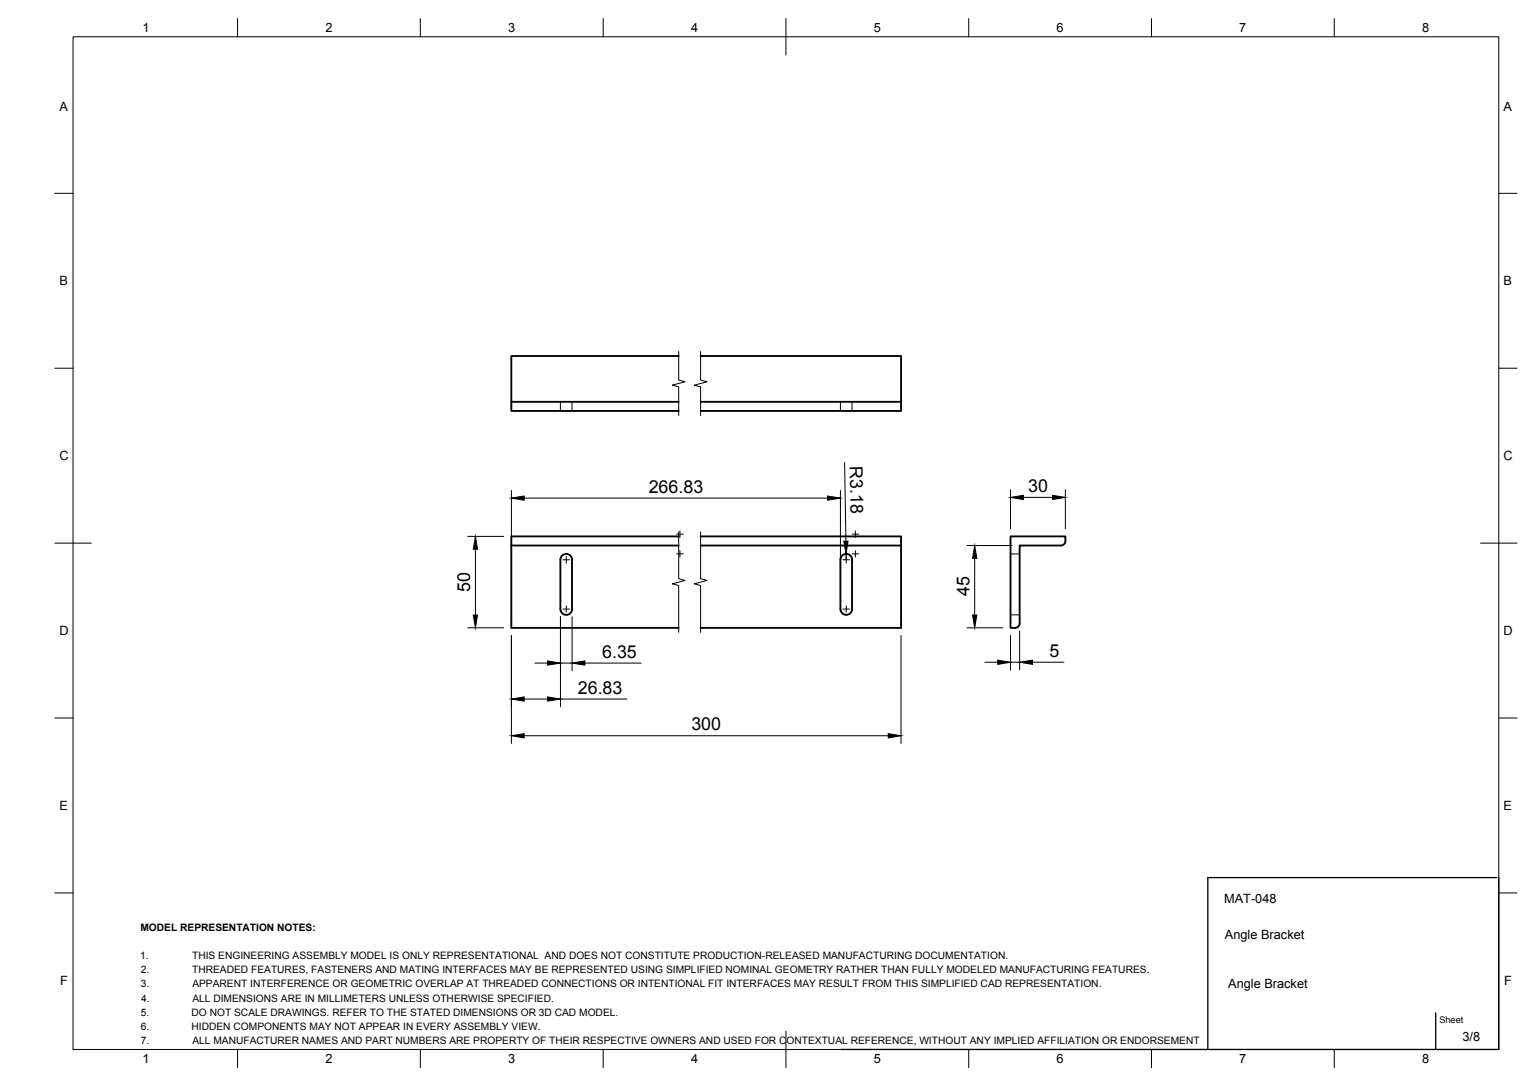
ISO-10303-21;
HEADER;
/* Generated by software containing ST-Developer
 * from STEP Tools, Inc. (www.steptools.com) 
 */

FILE_DESCRIPTION(
/* description */ ('STEP AP214'),
/* implementation_level */ '2;1');

FILE_NAME(
/* name */ 'Angle Bracket.step',
/* time_stamp */ '2026-11-14T22:24:45-08:00',
/* author */ (''),
/* organization */ (''),
/* preprocessor_version */ 'ST-DEVELOPER v20.2',
/* originating_system */ 'Autodesk Translation Framework v15.17.0.0',
/* authorisation */ '');

FILE_SCHEMA (('AUTOMOTIVE_DESIGN { 1 0 10303 214 3 1 1 }'));
ENDSEC;

DATA;
#10=MECHANICAL_DESIGN_GEOMETRIC_PRESENTATION_REPRESENTATION('',(#127),#5599);
#99=FACE_BOUND('',#563,.T.);
#100=FACE_BOUND('',#564,.T.);
#101=FACE_BOUND('',#570,.T.);
#102=FACE_BOUND('',#571,.T.);
#115=SHAPE_REPRESENTATION_RELATIONSHIP('SRR','None',#5643,#121);
#121=ADVANCED_BREP_SHAPE_REPRESENTATION('',(#133),#5595);
#127=STYLED_ITEM('',(#5681),#133);
#133=MANIFOLD_SOLID_BREP('Body1',#3309);
#165=CYLINDRICAL_SURFACE('',#3536,2.5);
#166=CYLINDRICAL_SURFACE('',#3545,2.5);
#167=CYLINDRICAL_SURFACE('',#3550,3.17499999999993);
#168=CYLINDRICAL_SURFACE('',#3552,3.17499999999993);
#169=CYLINDRICAL_SURFACE('',#3554,3.17499999999993);
#170=CYLINDRICAL_SURFACE('',#3556,3.17499999999993);
#225=CIRCLE('',#3530,3.17499999999993);
#226=CIRCLE('',#3531,3.17499999999993);
#227=CIRCLE('',#3532,3.17499999999993);
#228=CIRCLE('',#3533,3.17499999999993);
#229=CIRCLE('',#3537,2.5);
#230=CIRCLE('',#3538,2.5);
#231=CIRCLE('',#3541,3.17499999999993);
#232=CIRCLE('',#3542,3.17499999999993);
#233=CIRCLE('',#3543,3.17499999999993);
#234=CIRCLE('',#3544,3.17499999999993);
#235=CIRCLE('',#3546,2.5);
#236=CIRCLE('',#3547,2.5);
#385=FACE_OUTER_BOUND('',#561,.T.);
#386=FACE_OUTER_BOUND('',#562,.T.);
#387=FACE_OUTER_BOUND('',#565,.T.);
#388=FACE_OUTER_BOUND('',#566,.T.);
#389=FACE_OUTER_BOUND('',#567,.T.);
#390=FACE_OUTER_BOUND('',#568,.T.);
#391=FACE_OUTER_BOUND('',#569,.T.);
#392=FACE_OUTER_BOUND('',#572,.T.);
#393=FACE_OUTER_BOUND('',#573,.T.);
#394=FACE_OUTER_BOUND('',#574,.T.);
#395=FACE_OUTER_BOUND('',#575,.T.);
#396=FACE_OUTER_BOUND('',#576,.T.);
#397=FACE_OUTER_BOUND('',#577,.T.);
#398=FACE_OUTER_BOUND('',#578,.T.);
#399=FACE_OUTER_BOUND('',#579,.T.);
#400=FACE_OUTER_BOUND('',#580,.T.);
#401=FACE_OUTER_BOUND('',#581,.T.);
#402=FACE_OUTER_BOUND('',#582,.T.);
#561=EDGE_LOOP('',(#2635,#2636,#2637,#2638));
#562=EDGE_LOOP('',(#2639,#2640,#2641,#2642));
#563=EDGE_LOOP('',(#2643,#2644,#2645,#2646));
#564=EDGE_LOOP('',(#2647,#2648,#2649,#2650));
#565=EDGE_LOOP('',(#2651,#2652,#2653,#2654));
#566=EDGE_LOOP('',(#2655,#2656,#2657,#2658));
#567=EDGE_LOOP('',(#2659,#2660,#2661,#2662));
#568=EDGE_LOOP('',(#2663,#2664,#2665,#2666));
#569=EDGE_LOOP('',(#2667,#2668,#2669,#2670));
#570=EDGE_LOOP('',(#2671,#2672,#2673,#2674));
#571=EDGE_LOOP('',(#2675,#2676,#2677,#2678));
#572=EDGE_LOOP('',(#2679,#2680,#2681,#2682));
#573=EDGE_LOOP('',(#2683,#2684,#2685,#2686,#2687,#2688,#2689,#2690));
#574=EDGE_LOOP('',(#2691,#2692,#2693,#2694,#2695,#2696,#2697,#2698));
#575=EDGE_LOOP('',(#2699,#2700,#2701,#2702));
#576=EDGE_LOOP('',(#2703,#2704,#2705,#2706));
#577=EDGE_LOOP('',(#2707,#2708,#2709,#2710));
#578=EDGE_LOOP('',(#2711,#2712,#2713,#2714));
#579=EDGE_LOOP('',(#2715,#2716,#2717,#2718));
#580=EDGE_LOOP('',(#2719,#2720,#2721,#2722));
#581=EDGE_LOOP('',(#2723,#2724,#2725,#2726));
#582=EDGE_LOOP('',(#2727,#2728,#2729,#2730));
#875=LINE('',#5186,#1231);
#876=LINE('',#5188,#1232);
#877=LINE('',#5190,#1233);
#878=LINE('',#5191,#1234);
#879=LINE('',#5194,#1235);
#880=LINE('',#5196,#1236);
#881=LINE('',#5197,#1237);
#882=LINE('',#5200,#1238);
#883=LINE('',#5204,#1239);
#884=LINE('',#5208,#1240);
#885=LINE('',#5212,#1241);
#886=LINE('',#5216,#1242);
#887=LINE('',#5218,#1243);
#888=LINE('',#5219,#1244);
#889=LINE('',#5222,#1245);
#890=LINE('',#5224,#1246);
#891=LINE('',#5225,#1247);
#892=LINE('',#5230,#1248);
#893=LINE('',#5234,#1249);
#894=LINE('',#5236,#1250);
#895=LINE('',#5237,#1251);
#896=LINE('',#5240,#1252);
#897=LINE('',#5242,#1253);
#898=LINE('',#5243,#1254);
#899=LINE('',#5246,#1255);
#900=LINE('',#5250,#1256);
#901=LINE('',#5254,#1257);
#902=LINE('',#5258,#1258);
#903=LINE('',#5266,#1259);
#904=LINE('',#5267,#1260);
#905=LINE('',#5269,#1261);
#906=LINE('',#5271,#1262);
#907=LINE('',#5274,#1263);
#908=LINE('',#5275,#1264);
#909=LINE('',#5277,#1265);
#910=LINE('',#5279,#1266);
#1231=VECTOR('',#4207,1000.);
#1232=VECTOR('',#4208,1000.);
#1233=VECTOR('',#4209,1000.);
#1234=VECTOR('',#4210,1000.);
#1235=VECTOR('',#4213,1000.);
#1236=VECTOR('',#4214,1000.);
#1237=VECTOR('',#4215,1000.);
#1238=VECTOR('',#4216,1000.);
#1239=VECTOR('',#4219,1000.);
#1240=VECTOR('',#4222,1000.);
#1241=VECTOR('',#4225,1000.);
#1242=VECTOR('',#4230,1000.);
#1243=VECTOR('',#4231,1000.);
#1244=VECTOR('',#4232,1000.);
#1245=VECTOR('',#4235,1000.);
#1246=VECTOR('',#4236,1000.);
#1247=VECTOR('',#4237,1000.);
#1248=VECTOR('',#4242,1000.);
#1249=VECTOR('',#4247,1000.);
#1250=VECTOR('',#4248,1000.);
#1251=VECTOR('',#4249,1000.);
#1252=VECTOR('',#4252,1000.);
#1253=VECTOR('',#4253,1000.);
#1254=VECTOR('',#4254,1000.);
#1255=VECTOR('',#4255,1000.);
#1256=VECTOR('',#4258,1000.);
#1257=VECTOR('',#4261,1000.);
#1258=VECTOR('',#4264,1000.);
#1259=VECTOR('',#4279,1000.);
#1260=VECTOR('',#4280,1000.);
#1261=VECTOR('',#4283,1000.);
#1262=VECTOR('',#4286,1000.);
#1263=VECTOR('',#4291,1000.);
#1264=VECTOR('',#4292,1000.);
#1265=VECTOR('',#4295,1000.);
#1266=VECTOR('',#4298,1000.);
#1527=VERTEX_POINT('',#5184);
#1528=VERTEX_POINT('',#5185);
#1529=VERTEX_POINT('',#5187);
#1530=VERTEX_POINT('',#5189);
#1531=VERTEX_POINT('',#5193);
#1532=VERTEX_POINT('',#5195);
#1533=VERTEX_POINT('',#5198);
#1534=VERTEX_POINT('',#5199);
#1535=VERTEX_POINT('',#5201);
#1536=VERTEX_POINT('',#5203);
#1537=VERTEX_POINT('',#5206);
#1538=VERTEX_POINT('',#5207);
#1539=VERTEX_POINT('',#5209);
#1540=VERTEX_POINT('',#5211);
#1541=VERTEX_POINT('',#5215);
#1542=VERTEX_POINT('',#5217);
#1543=VERTEX_POINT('',#5221);
#1544=VERTEX_POINT('',#5223);
#1545=VERTEX_POINT('',#5227);
#1546=VERTEX_POINT('',#5229);
#1547=VERTEX_POINT('',#5233);
#1548=VERTEX_POINT('',#5235);
#1549=VERTEX_POINT('',#5239);
#1550=VERTEX_POINT('',#5241);
#1551=VERTEX_POINT('',#5244);
#1552=VERTEX_POINT('',#5245);
#1553=VERTEX_POINT('',#5247);
#1554=VERTEX_POINT('',#5249);
#1555=VERTEX_POINT('',#5252);
#1556=VERTEX_POINT('',#5253);
#1557=VERTEX_POINT('',#5255);
#1558=VERTEX_POINT('',#5257);
#1915=EDGE_CURVE('',#1527,#1528,#875,.T.);
#1916=EDGE_CURVE('',#1529,#1528,#876,.T.);
#1917=EDGE_CURVE('',#1530,#1529,#877,.T.);
#1918=EDGE_CURVE('',#1530,#1527,#878,.T.);
#1919=EDGE_CURVE('',#1528,#1531,#879,.T.);
#1920=EDGE_CURVE('',#1532,#1531,#880,.T.);
#1921=EDGE_CURVE('',#1529,#1532,#881,.T.);
#1922=EDGE_CURVE('',#1533,#1534,#882,.T.);
#1923=EDGE_CURVE('',#1534,#1535,#225,.T.);
#1924=EDGE_CURVE('',#1535,#1536,#883,.T.);
#1925=EDGE_CURVE('',#1536,#1533,#226,.T.);
#1926=EDGE_CURVE('',#1537,#1538,#884,.T.);
#1927=EDGE_CURVE('',#1538,#1539,#227,.T.);
#1928=EDGE_CURVE('',#1539,#1540,#885,.T.);
#1929=EDGE_CURVE('',#1540,#1537,#228,.T.);
#1930=EDGE_CURVE('',#1531,#1541,#886,.T.);
#1931=EDGE_CURVE('',#1542,#1541,#887,.T.);
#1932=EDGE_CURVE('',#1532,#1542,#888,.T.);
#1933=EDGE_CURVE('',#1541,#1543,#889,.T.);
#1934=EDGE_CURVE('',#1544,#1543,#890,.T.);
#1935=EDGE_CURVE('',#1542,#1544,#891,.T.);
#1936=EDGE_CURVE('',#1543,#1545,#229,.T.);
#1937=EDGE_CURVE('',#1546,#1545,#892,.T.);
#1938=EDGE_CURVE('',#1544,#1546,#230,.T.);
#1939=EDGE_CURVE('',#1545,#1547,#893,.T.);
#1940=EDGE_CURVE('',#1548,#1547,#894,.T.);
#1941=EDGE_CURVE('',#1546,#1548,#895,.T.);
#1942=EDGE_CURVE('',#1547,#1549,#896,.T.);
#1943=EDGE_CURVE('',#1550,#1549,#897,.T.);
#1944=EDGE_CURVE('',#1548,#1550,#898,.T.);
#1945=EDGE_CURVE('',#1551,#1552,#899,.T.);
#1946=EDGE_CURVE('',#1553,#1551,#231,.T.);
#1947=EDGE_CURVE('',#1554,#1553,#900,.T.);
#1948=EDGE_CURVE('',#1552,#1554,#232,.T.);
#1949=EDGE_CURVE('',#1555,#1556,#901,.T.);
#1950=EDGE_CURVE('',#1557,#1555,#233,.T.);
#1951=EDGE_CURVE('',#1558,#1557,#902,.T.);
#1952=EDGE_CURVE('',#1556,#1558,#234,.T.);
#1953=EDGE_CURVE('',#1549,#1527,#235,.T.);
#1954=EDGE_CURVE('',#1550,#1530,#236,.T.);
#1955=EDGE_CURVE('',#1538,#1557,#903,.T.);
#1956=EDGE_CURVE('',#1539,#1555,#904,.T.);
#1957=EDGE_CURVE('',#1537,#1558,#905,.T.);
#1958=EDGE_CURVE('',#1540,#1556,#906,.T.);
#1959=EDGE_CURVE('',#1534,#1553,#907,.T.);
#1960=EDGE_CURVE('',#1535,#1551,#908,.T.);
#1961=EDGE_CURVE('',#1533,#1554,#909,.T.);
#1962=EDGE_CURVE('',#1536,#1552,#910,.T.);
#2635=ORIENTED_EDGE('',*,*,#1915,.T.);
#2636=ORIENTED_EDGE('',*,*,#1916,.F.);
#2637=ORIENTED_EDGE('',*,*,#1917,.F.);
#2638=ORIENTED_EDGE('',*,*,#1918,.T.);
#2639=ORIENTED_EDGE('',*,*,#1919,.T.);
#2640=ORIENTED_EDGE('',*,*,#1920,.F.);
#2641=ORIENTED_EDGE('',*,*,#1921,.F.);
#2642=ORIENTED_EDGE('',*,*,#1916,.T.);
#2643=ORIENTED_EDGE('',*,*,#1922,.T.);
#2644=ORIENTED_EDGE('',*,*,#1923,.T.);
#2645=ORIENTED_EDGE('',*,*,#1924,.T.);
#2646=ORIENTED_EDGE('',*,*,#1925,.T.);
#2647=ORIENTED_EDGE('',*,*,#1926,.T.);
#2648=ORIENTED_EDGE('',*,*,#1927,.T.);
#2649=ORIENTED_EDGE('',*,*,#1928,.T.);
#2650=ORIENTED_EDGE('',*,*,#1929,.T.);
#2651=ORIENTED_EDGE('',*,*,#1930,.T.);
#2652=ORIENTED_EDGE('',*,*,#1931,.F.);
#2653=ORIENTED_EDGE('',*,*,#1932,.F.);
#2654=ORIENTED_EDGE('',*,*,#1920,.T.);
#2655=ORIENTED_EDGE('',*,*,#1933,.T.);
#2656=ORIENTED_EDGE('',*,*,#1934,.F.);
#2657=ORIENTED_EDGE('',*,*,#1935,.F.);
#2658=ORIENTED_EDGE('',*,*,#1931,.T.);
#2659=ORIENTED_EDGE('',*,*,#1936,.T.);
#2660=ORIENTED_EDGE('',*,*,#1937,.F.);
#2661=ORIENTED_EDGE('',*,*,#1938,.F.);
#2662=ORIENTED_EDGE('',*,*,#1934,.T.);
#2663=ORIENTED_EDGE('',*,*,#1939,.T.);
#2664=ORIENTED_EDGE('',*,*,#1940,.F.);
#2665=ORIENTED_EDGE('',*,*,#1941,.F.);
#2666=ORIENTED_EDGE('',*,*,#1937,.T.);
#2667=ORIENTED_EDGE('',*,*,#1942,.T.);
#2668=ORIENTED_EDGE('',*,*,#1943,.F.);
#2669=ORIENTED_EDGE('',*,*,#1944,.F.);
#2670=ORIENTED_EDGE('',*,*,#1940,.T.);
#2671=ORIENTED_EDGE('',*,*,#1945,.F.);
#2672=ORIENTED_EDGE('',*,*,#1946,.F.);
#2673=ORIENTED_EDGE('',*,*,#1947,.F.);
#2674=ORIENTED_EDGE('',*,*,#1948,.F.);
#2675=ORIENTED_EDGE('',*,*,#1949,.F.);
#2676=ORIENTED_EDGE('',*,*,#1950,.F.);
#2677=ORIENTED_EDGE('',*,*,#1951,.F.);
#2678=ORIENTED_EDGE('',*,*,#1952,.F.);
#2679=ORIENTED_EDGE('',*,*,#1953,.T.);
#2680=ORIENTED_EDGE('',*,*,#1918,.F.);
#2681=ORIENTED_EDGE('',*,*,#1954,.F.);
#2682=ORIENTED_EDGE('',*,*,#1943,.T.);
#2683=ORIENTED_EDGE('',*,*,#1917,.T.);
#2684=ORIENTED_EDGE('',*,*,#1921,.T.);
#2685=ORIENTED_EDGE('',*,*,#1932,.T.);
#2686=ORIENTED_EDGE('',*,*,#1935,.T.);
#2687=ORIENTED_EDGE('',*,*,#1938,.T.);
#2688=ORIENTED_EDGE('',*,*,#1941,.T.);
#2689=ORIENTED_EDGE('',*,*,#1944,.T.);
#2690=ORIENTED_EDGE('',*,*,#1954,.T.);
#2691=ORIENTED_EDGE('',*,*,#1915,.F.);
#2692=ORIENTED_EDGE('',*,*,#1953,.F.);
#2693=ORIENTED_EDGE('',*,*,#1942,.F.);
#2694=ORIENTED_EDGE('',*,*,#1939,.F.);
#2695=ORIENTED_EDGE('',*,*,#1936,.F.);
#2696=ORIENTED_EDGE('',*,*,#1933,.F.);
#2697=ORIENTED_EDGE('',*,*,#1930,.F.);
#2698=ORIENTED_EDGE('',*,*,#1919,.F.);
#2699=ORIENTED_EDGE('',*,*,#1955,.T.);
#2700=ORIENTED_EDGE('',*,*,#1950,.T.);
#2701=ORIENTED_EDGE('',*,*,#1956,.F.);
#2702=ORIENTED_EDGE('',*,*,#1927,.F.);
#2703=ORIENTED_EDGE('',*,*,#1957,.T.);
#2704=ORIENTED_EDGE('',*,*,#1951,.T.);
#2705=ORIENTED_EDGE('',*,*,#1955,.F.);
#2706=ORIENTED_EDGE('',*,*,#1926,.F.);
#2707=ORIENTED_EDGE('',*,*,#1958,.T.);
#2708=ORIENTED_EDGE('',*,*,#1952,.T.);
#2709=ORIENTED_EDGE('',*,*,#1957,.F.);
#2710=ORIENTED_EDGE('',*,*,#1929,.F.);
#2711=ORIENTED_EDGE('',*,*,#1956,.T.);
#2712=ORIENTED_EDGE('',*,*,#1949,.T.);
#2713=ORIENTED_EDGE('',*,*,#1958,.F.);
#2714=ORIENTED_EDGE('',*,*,#1928,.F.);
#2715=ORIENTED_EDGE('',*,*,#1959,.T.);
#2716=ORIENTED_EDGE('',*,*,#1946,.T.);
#2717=ORIENTED_EDGE('',*,*,#1960,.F.);
#2718=ORIENTED_EDGE('',*,*,#1923,.F.);
#2719=ORIENTED_EDGE('',*,*,#1961,.T.);
#2720=ORIENTED_EDGE('',*,*,#1947,.T.);
#2721=ORIENTED_EDGE('',*,*,#1959,.F.);
#2722=ORIENTED_EDGE('',*,*,#1922,.F.);
#2723=ORIENTED_EDGE('',*,*,#1962,.T.);
#2724=ORIENTED_EDGE('',*,*,#1948,.T.);
#2725=ORIENTED_EDGE('',*,*,#1961,.F.);
#2726=ORIENTED_EDGE('',*,*,#1925,.F.);
#2727=ORIENTED_EDGE('',*,*,#1960,.T.);
#2728=ORIENTED_EDGE('',*,*,#1945,.T.);
#2729=ORIENTED_EDGE('',*,*,#1962,.F.);
#2730=ORIENTED_EDGE('',*,*,#1924,.F.);
#3087=PLANE('',#3528);
#3088=PLANE('',#3529);
#3089=PLANE('',#3534);
#3090=PLANE('',#3535);
#3091=PLANE('',#3539);
#3092=PLANE('',#3540);
#3093=PLANE('',#3548);
#3094=PLANE('',#3549);
#3095=PLANE('',#3551);
#3096=PLANE('',#3553);
#3097=PLANE('',#3555);
#3098=PLANE('',#3557);
#3235=ADVANCED_FACE('',(#385),#3087,.F.);
#3236=ADVANCED_FACE('',(#386,#99,#100),#3088,.F.);
#3237=ADVANCED_FACE('',(#387),#3089,.F.);
#3238=ADVANCED_FACE('',(#388),#3090,.F.);
#3239=ADVANCED_FACE('',(#389),#165,.T.);
#3240=ADVANCED_FACE('',(#390),#3091,.F.);
#3241=ADVANCED_FACE('',(#391,#101,#102),#3092,.F.);
#3242=ADVANCED_FACE('',(#392),#166,.T.);
#3243=ADVANCED_FACE('',(#393),#3093,.T.);
#3244=ADVANCED_FACE('',(#394),#3094,.F.);
#3245=ADVANCED_FACE('',(#395),#167,.F.);
#3246=ADVANCED_FACE('',(#396),#3095,.F.);
#3247=ADVANCED_FACE('',(#397),#168,.F.);
#3248=ADVANCED_FACE('',(#398),#3096,.F.);
#3249=ADVANCED_FACE('',(#399),#169,.F.);
#3250=ADVANCED_FACE('',(#400),#3097,.F.);
#3251=ADVANCED_FACE('',(#401),#170,.F.);
#3252=ADVANCED_FACE('',(#402),#3098,.F.);
#3309=CLOSED_SHELL('',(#3235,#3236,#3237,#3238,#3239,#3240,#3241,#3242,
#3243,#3244,#3245,#3246,#3247,#3248,#3249,#3250,#3251,#3252));
#3527=AXIS2_PLACEMENT_3D('',#5182,#4203,#4204);
#3528=AXIS2_PLACEMENT_3D('',#5183,#4205,#4206);
#3529=AXIS2_PLACEMENT_3D('',#5192,#4211,#4212);
#3530=AXIS2_PLACEMENT_3D('',#5202,#4217,#4218);
#3531=AXIS2_PLACEMENT_3D('',#5205,#4220,#4221);
#3532=AXIS2_PLACEMENT_3D('',#5210,#4223,#4224);
#3533=AXIS2_PLACEMENT_3D('',#5213,#4226,#4227);
#3534=AXIS2_PLACEMENT_3D('',#5214,#4228,#4229);
#3535=AXIS2_PLACEMENT_3D('',#5220,#4233,#4234);
#3536=AXIS2_PLACEMENT_3D('',#5226,#4238,#4239);
#3537=AXIS2_PLACEMENT_3D('',#5228,#4240,#4241);
#3538=AXIS2_PLACEMENT_3D('',#5231,#4243,#4244);
#3539=AXIS2_PLACEMENT_3D('',#5232,#4245,#4246);
#3540=AXIS2_PLACEMENT_3D('',#5238,#4250,#4251);
#3541=AXIS2_PLACEMENT_3D('',#5248,#4256,#4257);
#3542=AXIS2_PLACEMENT_3D('',#5251,#4259,#4260);
#3543=AXIS2_PLACEMENT_3D('',#5256,#4262,#4263);
#3544=AXIS2_PLACEMENT_3D('',#5259,#4265,#4266);
#3545=AXIS2_PLACEMENT_3D('',#5260,#4267,#4268);
#3546=AXIS2_PLACEMENT_3D('',#5261,#4269,#4270);
#3547=AXIS2_PLACEMENT_3D('',#5262,#4271,#4272);
#3548=AXIS2_PLACEMENT_3D('',#5263,#4273,#4274);
#3549=AXIS2_PLACEMENT_3D('',#5264,#4275,#4276);
#3550=AXIS2_PLACEMENT_3D('',#5265,#4277,#4278);
#3551=AXIS2_PLACEMENT_3D('',#5268,#4281,#4282);
#3552=AXIS2_PLACEMENT_3D('',#5270,#4284,#4285);
#3553=AXIS2_PLACEMENT_3D('',#5272,#4287,#4288);
#3554=AXIS2_PLACEMENT_3D('',#5273,#4289,#4290);
#3555=AXIS2_PLACEMENT_3D('',#5276,#4293,#4294);
#3556=AXIS2_PLACEMENT_3D('',#5278,#4296,#4297);
#3557=AXIS2_PLACEMENT_3D('',#5280,#4299,#4300);
#4203=DIRECTION('axis',(0.,0.,1.));
#4204=DIRECTION('refdir',(1.,0.,0.));
#4205=DIRECTION('center_axis',(1.,0.,0.));
#4206=DIRECTION('ref_axis',(0.,0.,-1.));
#4207=DIRECTION('',(0.,-1.,0.));
#4208=DIRECTION('',(0.,0.,-1.));
#4209=DIRECTION('',(0.,-1.,0.));
#4210=DIRECTION('',(0.,0.,-1.));
#4211=DIRECTION('center_axis',(0.,1.,0.));
#4212=DIRECTION('ref_axis',(0.,0.,1.));
#4213=DIRECTION('',(1.,0.,0.));
#4214=DIRECTION('',(0.,0.,-1.));
#4215=DIRECTION('',(1.,0.,0.));
#4216=DIRECTION('',(-1.,0.,1.28577838368676E-16));
#4217=DIRECTION('center_axis',(0.,1.,0.));
#4218=DIRECTION('ref_axis',(0.,0.,1.));
#4219=DIRECTION('',(1.,0.,0.));
#4220=DIRECTION('center_axis',(0.,1.,0.));
#4221=DIRECTION('ref_axis',(0.,0.,1.));
#4222=DIRECTION('',(-1.,0.,0.));
#4223=DIRECTION('center_axis',(0.,1.,0.));
#4224=DIRECTION('ref_axis',(0.,0.,1.));
#4225=DIRECTION('',(1.,0.,0.));
#4226=DIRECTION('center_axis',(0.,1.,0.));
#4227=DIRECTION('ref_axis',(0.,0.,1.));
#4228=DIRECTION('center_axis',(-1.,0.,0.));
#4229=DIRECTION('ref_axis',(0.,0.,1.));
#4230=DIRECTION('',(0.,1.,0.));
#4231=DIRECTION('',(0.,0.,-1.));
#4232=DIRECTION('',(0.,1.,0.));
#4233=DIRECTION('center_axis',(0.,-1.,0.));
#4234=DIRECTION('ref_axis',(0.,0.,-1.));
#4235=DIRECTION('',(-1.,0.,0.));
#4236=DIRECTION('',(0.,0.,-1.));
#4237=DIRECTION('',(-1.,0.,0.));
#4238=DIRECTION('center_axis',(0.,0.,-1.));
#4239=DIRECTION('ref_axis',(-1.,0.,0.));
#4240=DIRECTION('center_axis',(0.,0.,1.));
#4241=DIRECTION('ref_axis',(-1.,0.,0.));
#4242=DIRECTION('',(0.,0.,-1.));
#4243=DIRECTION('center_axis',(0.,0.,1.));
#4244=DIRECTION('ref_axis',(-1.,0.,0.));
#4245=DIRECTION('center_axis',(1.,0.,0.));
#4246=DIRECTION('ref_axis',(0.,0.,-1.));
#4247=DIRECTION('',(0.,-1.,0.));
#4248=DIRECTION('',(0.,0.,-1.));
#4249=DIRECTION('',(0.,-1.,0.));
#4250=DIRECTION('center_axis',(0.,-1.,0.));
#4251=DIRECTION('ref_axis',(0.,0.,-1.));
#4252=DIRECTION('',(-1.,0.,0.));
#4253=DIRECTION('',(0.,0.,-1.));
#4254=DIRECTION('',(-1.,0.,0.));
#4255=DIRECTION('',(1.,0.,0.));
#4256=DIRECTION('center_axis',(0.,1.,0.));
#4257=DIRECTION('ref_axis',(0.,0.,1.));
#4258=DIRECTION('',(-1.,0.,1.28577838368676E-16));
#4259=DIRECTION('center_axis',(0.,1.,0.));
#4260=DIRECTION('ref_axis',(0.,0.,1.));
#4261=DIRECTION('',(1.,0.,0.));
#4262=DIRECTION('center_axis',(0.,1.,0.));
#4263=DIRECTION('ref_axis',(0.,0.,-1.));
#4264=DIRECTION('',(-1.,0.,0.));
#4265=DIRECTION('center_axis',(0.,1.,0.));
#4266=DIRECTION('ref_axis',(0.,0.,-1.));
#4267=DIRECTION('center_axis',(0.,0.,-1.));
#4268=DIRECTION('ref_axis',(-1.,0.,0.));
#4269=DIRECTION('center_axis',(0.,0.,1.));
#4270=DIRECTION('ref_axis',(1.,0.,0.));
#4271=DIRECTION('center_axis',(0.,0.,1.));
#4272=DIRECTION('ref_axis',(1.,0.,0.));
#4273=DIRECTION('center_axis',(0.,0.,1.));
#4274=DIRECTION('ref_axis',(1.,0.,0.));
#4275=DIRECTION('center_axis',(0.,0.,1.));
#4276=DIRECTION('ref_axis',(1.,0.,0.));
#4277=DIRECTION('center_axis',(0.,1.,0.));
#4278=DIRECTION('ref_axis',(0.,0.,1.));
#4279=DIRECTION('',(0.,1.,0.));
#4280=DIRECTION('',(0.,1.,0.));
#4281=DIRECTION('center_axis',(0.,0.,-1.));
#4282=DIRECTION('ref_axis',(-1.,0.,0.));
#4283=DIRECTION('',(0.,1.,0.));
#4284=DIRECTION('center_axis',(0.,1.,0.));
#4285=DIRECTION('ref_axis',(0.,0.,1.));
#4286=DIRECTION('',(0.,1.,0.));
#4287=DIRECTION('center_axis',(0.,0.,1.));
#4288=DIRECTION('ref_axis',(1.,0.,0.));
#4289=DIRECTION('center_axis',(0.,1.,0.));
#4290=DIRECTION('ref_axis',(0.,0.,1.));
#4291=DIRECTION('',(0.,1.,0.));
#4292=DIRECTION('',(0.,1.,0.));
#4293=DIRECTION('center_axis',(-1.28577838368676E-16,0.,-1.));
#4294=DIRECTION('ref_axis',(-1.,0.,1.28577838368676E-16));
#4295=DIRECTION('',(0.,1.,0.));
#4296=DIRECTION('center_axis',(0.,1.,0.));
#4297=DIRECTION('ref_axis',(0.,0.,1.));
#4298=DIRECTION('',(0.,1.,0.));
#4299=DIRECTION('center_axis',(0.,0.,1.));
#4300=DIRECTION('ref_axis',(1.,0.,0.));
#5182=CARTESIAN_POINT('',(0.,0.,0.));
#5183=CARTESIAN_POINT('Origin',(-5.55111512312578E-14,0.,300.));
#5184=CARTESIAN_POINT('',(0.,2.49999999999998,0.));
#5185=CARTESIAN_POINT('',(0.,0.,0.));
#5186=CARTESIAN_POINT('',(0.,0.,0.));
#5187=CARTESIAN_POINT('',(-5.55111512312578E-14,0.,300.));
#5188=CARTESIAN_POINT('',(-5.55111512312578E-14,0.,300.));
#5189=CARTESIAN_POINT('',(-5.55111512312578E-14,2.49999999999998,300.));
#5190=CARTESIAN_POINT('',(-5.55111512312578E-14,0.,300.));
#5191=CARTESIAN_POINT('',(-5.55111512312578E-14,2.49999999999998,300.));
#5192=CARTESIAN_POINT('Origin',(-5.55111512312578E-14,0.,300.));
#5193=CARTESIAN_POINT('',(50.,0.,-5.55111512312578E-14));
#5194=CARTESIAN_POINT('',(0.,0.,0.));
#5195=CARTESIAN_POINT('',(50.,0.,300.));
#5196=CARTESIAN_POINT('',(50.,0.,300.));
#5197=CARTESIAN_POINT('',(-5.55111512312578E-14,0.,300.));
#5198=CARTESIAN_POINT('',(37.2416210910529,-5.55111512312578E-14,26.825));
#5199=CARTESIAN_POINT('',(10.2583789089471,-5.55111512312578E-14,26.825));
#5200=CARTESIAN_POINT('',(-2.77555756156289E-14,0.,26.825));
#5201=CARTESIAN_POINT('',(10.2583789089471,-5.55111512312578E-14,33.1749999999999));
#5202=CARTESIAN_POINT('Origin',(10.2583789089471,0.,29.9999999999999));
#5203=CARTESIAN_POINT('',(37.2416210910529,0.,33.1749999999999));
#5204=CARTESIAN_POINT('',(-5.55111512312578E-14,0.,33.1749999999999));
#5205=CARTESIAN_POINT('Origin',(37.2416210910529,0.,30.));
#5206=CARTESIAN_POINT('',(37.2416210910529,-5.55111512312578E-14,266.825));
#5207=CARTESIAN_POINT('',(10.2583789089472,-5.55111512312578E-14,266.825));
#5208=CARTESIAN_POINT('',(0.,0.,266.825));
#5209=CARTESIAN_POINT('',(10.2583789089472,-5.55111512312578E-14,273.175));
#5210=CARTESIAN_POINT('Origin',(10.2583789089472,0.,270.));
#5211=CARTESIAN_POINT('',(37.2416210910529,0.,273.175));
#5212=CARTESIAN_POINT('',(0.,0.,273.175));
#5213=CARTESIAN_POINT('Origin',(37.2416210910529,0.,270.));
#5214=CARTESIAN_POINT('Origin',(50.,0.,300.));
#5215=CARTESIAN_POINT('',(50.,30.,-5.55111512312578E-14));
#5216=CARTESIAN_POINT('',(50.,0.,-5.55111512312578E-14));
#5217=CARTESIAN_POINT('',(50.,30.,300.));
#5218=CARTESIAN_POINT('',(50.,30.,300.));
#5219=CARTESIAN_POINT('',(50.,0.,300.));
#5220=CARTESIAN_POINT('Origin',(50.,30.,300.));
#5221=CARTESIAN_POINT('',(47.5,30.,0.));
#5222=CARTESIAN_POINT('',(50.,30.,-5.55111512312578E-14));
#5223=CARTESIAN_POINT('',(47.5,30.,300.));
#5224=CARTESIAN_POINT('',(47.5,30.,300.));
#5225=CARTESIAN_POINT('',(50.,30.,300.));
#5226=CARTESIAN_POINT('Origin',(47.5,27.5,300.));
#5227=CARTESIAN_POINT('',(45.,27.5,0.));
#5228=CARTESIAN_POINT('Origin',(47.5,27.5,0.));
#5229=CARTESIAN_POINT('',(45.,27.5,300.));
#5230=CARTESIAN_POINT('',(45.,27.5,300.));
#5231=CARTESIAN_POINT('Origin',(47.5,27.5,300.));
#5232=CARTESIAN_POINT('Origin',(45.,5.,300.));
#5233=CARTESIAN_POINT('',(45.,5.,0.));
#5234=CARTESIAN_POINT('',(45.,5.,0.));
#5235=CARTESIAN_POINT('',(45.,5.,300.));
#5236=CARTESIAN_POINT('',(45.,5.,300.));
#5237=CARTESIAN_POINT('',(45.,5.,300.));
#5238=CARTESIAN_POINT('Origin',(2.49999999999997,5.,300.));
#5239=CARTESIAN_POINT('',(2.50000000000003,5.,-5.55111512312578E-14));
#5240=CARTESIAN_POINT('',(2.50000000000003,5.,-5.55111512312578E-14));
#5241=CARTESIAN_POINT('',(2.49999999999997,5.,300.));
#5242=CARTESIAN_POINT('',(2.49999999999997,5.,300.));
#5243=CARTESIAN_POINT('',(2.49999999999997,5.,300.));
#5244=CARTESIAN_POINT('',(10.2583789089471,5.,33.1749999999999));
#5245=CARTESIAN_POINT('',(37.2416210910529,5.,33.1749999999999));
#5246=CARTESIAN_POINT('',(10.2583789089471,5.,33.1749999999999));
#5247=CARTESIAN_POINT('',(10.2583789089471,5.,26.825));
#5248=CARTESIAN_POINT('Origin',(10.2583789089471,5.,29.9999999999999));
#5249=CARTESIAN_POINT('',(37.2416210910529,5.,26.825));
#5250=CARTESIAN_POINT('',(10.2583789089471,5.,26.825));
#5251=CARTESIAN_POINT('Origin',(37.2416210910529,5.,30.));
#5252=CARTESIAN_POINT('',(10.2583789089472,5.,273.175));
#5253=CARTESIAN_POINT('',(37.2416210910529,5.,273.175));
#5254=CARTESIAN_POINT('',(10.2583789089472,5.,273.175));
#5255=CARTESIAN_POINT('',(10.2583789089472,5.,266.825));
#5256=CARTESIAN_POINT('Origin',(10.2583789089472,5.,270.));
#5257=CARTESIAN_POINT('',(37.2416210910529,5.,266.825));
#5258=CARTESIAN_POINT('',(10.2583789089472,5.,266.825));
#5259=CARTESIAN_POINT('Origin',(37.2416210910529,5.,270.));
#5260=CARTESIAN_POINT('Origin',(2.49999999999995,2.5,300.));
#5261=CARTESIAN_POINT('Origin',(2.5,2.5,-5.55111512312578E-14));
#5262=CARTESIAN_POINT('Origin',(2.49999999999995,2.5,300.));
#5263=CARTESIAN_POINT('Origin',(2.49999999999995,2.5,300.));
#5264=CARTESIAN_POINT('Origin',(2.5,2.5,-5.55111512312578E-14));
#5265=CARTESIAN_POINT('Origin',(10.2583789089472,-175.,270.));
#5266=CARTESIAN_POINT('',(10.2583789089472,-175.,266.825));
#5267=CARTESIAN_POINT('',(10.2583789089472,-175.,273.175));
#5268=CARTESIAN_POINT('Origin',(10.2583789089472,-175.,266.825));
#5269=CARTESIAN_POINT('',(37.2416210910529,-175.,266.825));
#5270=CARTESIAN_POINT('Origin',(37.2416210910529,-175.,270.));
#5271=CARTESIAN_POINT('',(37.2416210910529,-175.,273.175));
#5272=CARTESIAN_POINT('Origin',(10.2583789089472,-175.,273.175));
#5273=CARTESIAN_POINT('Origin',(10.2583789089471,-175.,29.9999999999999));
#5274=CARTESIAN_POINT('',(10.2583789089471,-175.,26.825));
#5275=CARTESIAN_POINT('',(10.2583789089471,-175.,33.1749999999999));
#5276=CARTESIAN_POINT('Origin',(10.2583789089471,-175.,26.825));
#5277=CARTESIAN_POINT('',(37.2416210910529,-175.,26.825));
#5278=CARTESIAN_POINT('Origin',(37.2416210910529,-175.,30.));
#5279=CARTESIAN_POINT('',(37.2416210910529,-175.,33.1749999999999));
#5280=CARTESIAN_POINT('Origin',(10.2583789089471,-175.,33.1749999999999));
#5587=UNCERTAINTY_MEASURE_WITH_UNIT(LENGTH_MEASURE(0.01),#5600,
'DISTANCE_ACCURACY_VALUE',
'Maximum model space distance between geometric entities at asserted c
onnectivities');
#5591=UNCERTAINTY_MEASURE_WITH_UNIT(LENGTH_MEASURE(0.01),#5600,
'DISTANCE_ACCURACY_VALUE',
'Maximum model space distance between geometric entities at asserted c
onnectivities');
#5595=(
GEOMETRIC_REPRESENTATION_CONTEXT(3)
GLOBAL_UNCERTAINTY_ASSIGNED_CONTEXT((#5587))
GLOBAL_UNIT_ASSIGNED_CONTEXT((#5600,#5602,#5603))
REPRESENTATION_CONTEXT('','3D')
);
#5599=(
GEOMETRIC_REPRESENTATION_CONTEXT(3)
GLOBAL_UNCERTAINTY_ASSIGNED_CONTEXT((#5591))
GLOBAL_UNIT_ASSIGNED_CONTEXT((#5600,#5602,#5603))
REPRESENTATION_CONTEXT('','3D')
);
#5600=(
LENGTH_UNIT()
NAMED_UNIT(*)
SI_UNIT(.MILLI.,.METRE.)
);
#5602=(
NAMED_UNIT(*)
PLANE_ANGLE_UNIT()
SI_UNIT($,.RADIAN.)
);
#5603=(
NAMED_UNIT(*)
SI_UNIT($,.STERADIAN.)
SOLID_ANGLE_UNIT()
);
#5607=SHAPE_DEFINITION_REPRESENTATION(#5614,#5643);
#5614=PRODUCT_DEFINITION_SHAPE('',$,#5651);
#5643=SHAPE_REPRESENTATION('',(#3527),#5595);
#5647=PRODUCT_DEFINITION_CONTEXT('part definition',#5670,'design');
#5651=PRODUCT_DEFINITION('Angle Bracket','Angle Bracket',#5658,#5647);
#5658=PRODUCT_DEFINITION_FORMATION('',$,#5675);
#5670=APPLICATION_CONTEXT(
'Core Data for Automotive Mechanical Design Process');
#5671=PRODUCT_CONTEXT('part definition',#5670,'mechanical');
#5675=PRODUCT('Angle Bracket','Angle Bracket',$,(#5671));
#5681=PRESENTATION_STYLE_ASSIGNMENT((#5684));
#5684=SURFACE_STYLE_USAGE(.BOTH.,#5687);
#5687=SURFACE_SIDE_STYLE('',(#5690));
#5690=SURFACE_STYLE_FILL_AREA(#5693);
#5693=FILL_AREA_STYLE('Opaque(227,224,212)',(#5696));
#5696=FILL_AREA_STYLE_COLOUR('Opaque(227,224,212)',#5699);
#5699=COLOUR_RGB('Opaque(227,224,212)',0.890196078431372,0.87843137254902,
0.831372549019608);
ENDSEC;
END-ISO-10303-21;
